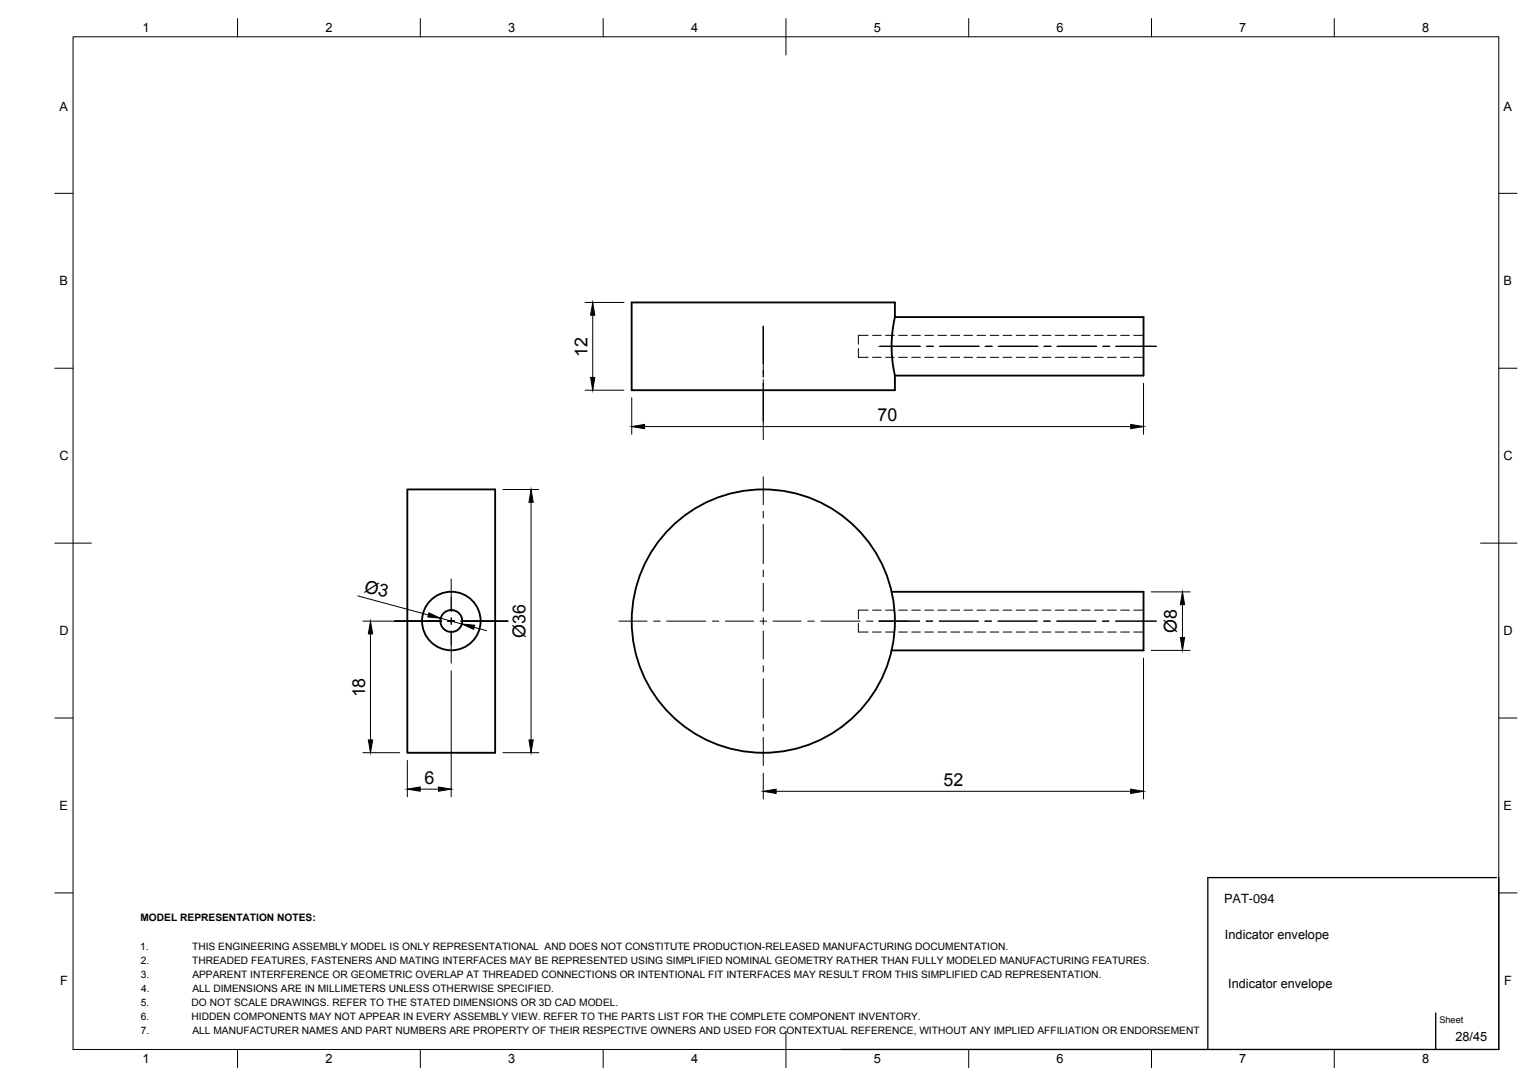
ISO-10303-21;
HEADER;
/* Generated by software containing ST-Developer
 * from STEP Tools, Inc. (www.steptools.com) 
 */

FILE_DESCRIPTION(
/* description */ ('Shaft runout checking stand'),
/* implementation_level */ '2;1');

FILE_NAME(
/* name */ 'Indicator envelope.step',
/* time_stamp */ '2026-11-02T21:12:33-08:00',
/* author */ (''),
/* organization */ (''),
/* preprocessor_version */ 'ST-DEVELOPER v20.2',
/* originating_system */ 'Autodesk Translation Framework v15.17.0.0',
/* authorisation */ '');

FILE_SCHEMA (('AUTOMOTIVE_DESIGN { 1 0 10303 214 3 1 1 }'));
ENDSEC;

DATA;
#10=MECHANICAL_DESIGN_GEOMETRIC_PRESENTATION_REPRESENTATION('',(#490),#11748);
#333=B_SPLINE_CURVE_WITH_KNOTS('',3,(#10807,#10808,#10809,#10810,#10811,
#10812,#10813,#10814,#10815,#10816,#10817,#10818,#10819,#10820,#10821,#10822,
#10823,#10824),.UNSPECIFIED.,.F.,.F.,(4,2,2,2,2,2,2,2,4),(0.,0.151225950236217,
0.302451900472435,0.453664817813398,0.604877735154361,0.756090652495325,
0.907303569836288,1.05852952007251,1.20975547030872),.UNSPECIFIED.);
#334=B_SPLINE_CURVE_WITH_KNOTS('',3,(#10825,#10826,#10827,#10828,#10829,
#10830,#10831,#10832,#10833,#10834,#10835,#10836,#10837,#10838,#10839,#10840,
#10841,#10842),.UNSPECIFIED.,.F.,.F.,(4,2,2,2,2,2,2,2,4),(1.20975547030872,
1.36098142054494,1.51220737078116,1.66342028812212,1.81463320546308,1.96584612280405,
2.11705904014501,2.26828499038123,2.41951094061745),.UNSPECIFIED.);
#404=SHAPE_REPRESENTATION_RELATIONSHIP('SRR','None',#11953,#447);
#447=ADVANCED_BREP_SHAPE_REPRESENTATION('',(#538),#11729);
#490=STYLED_ITEM('',(#12169),#538);
#538=MANIFOLD_SOLID_BREP('Body1',#6236);
#650=FACE_BOUND('',#1770,.T.);
#651=FACE_BOUND('',#1772,.T.);
#831=CIRCLE('',#7197,0.15);
#832=CIRCLE('',#7198,0.15);
#833=CIRCLE('',#7201,0.4);
#834=CIRCLE('',#7204,1.8);
#835=CIRCLE('',#7205,1.8);
#1008=CYLINDRICAL_SURFACE('',#7196,0.15);
#1009=CYLINDRICAL_SURFACE('',#7200,0.4);
#1010=CYLINDRICAL_SURFACE('',#7203,1.8);
#1310=FACE_OUTER_BOUND('',#1766,.T.);
#1311=FACE_OUTER_BOUND('',#1767,.T.);
#1312=FACE_OUTER_BOUND('',#1768,.T.);
#1313=FACE_OUTER_BOUND('',#1769,.T.);
#1314=FACE_OUTER_BOUND('',#1771,.T.);
#1315=FACE_OUTER_BOUND('',#1773,.T.);
#1316=FACE_OUTER_BOUND('',#1774,.T.);
#1766=EDGE_LOOP('',(#5264,#5265,#5266,#5267));
#1767=EDGE_LOOP('',(#5268));
#1768=EDGE_LOOP('',(#5269,#5270,#5271,#5272,#5273));
#1769=EDGE_LOOP('',(#5274));
#1770=EDGE_LOOP('',(#5275));
#1771=EDGE_LOOP('',(#5276,#5277,#5278,#5279));
#1772=EDGE_LOOP('',(#5280,#5281));
#1773=EDGE_LOOP('',(#5282));
#1774=EDGE_LOOP('',(#5283));
#2309=LINE('',#10801,#2776);
#2310=LINE('',#10844,#2777);
#2311=LINE('',#10851,#2778);
#2776=VECTOR('',#8844,0.15);
#2777=VECTOR('',#8851,0.4);
#2778=VECTOR('',#8860,1.8);
#3207=VERTEX_POINT('',#10798);
#3208=VERTEX_POINT('',#10800);
#3209=VERTEX_POINT('',#10805);
#3210=VERTEX_POINT('',#10806);
#3211=VERTEX_POINT('',#10843);
#3212=VERTEX_POINT('',#10848);
#3213=VERTEX_POINT('',#10850);
#3918=EDGE_CURVE('',#3207,#3207,#831,.T.);
#3919=EDGE_CURVE('',#3207,#3208,#2309,.T.);
#3920=EDGE_CURVE('',#3208,#3208,#832,.T.);
#3921=EDGE_CURVE('',#3209,#3210,#333,.T.);
#3922=EDGE_CURVE('',#3210,#3209,#334,.T.);
#3923=EDGE_CURVE('',#3210,#3211,#2310,.T.);
#3924=EDGE_CURVE('',#3211,#3211,#833,.T.);
#3925=EDGE_CURVE('',#3212,#3212,#834,.T.);
#3926=EDGE_CURVE('',#3212,#3213,#2311,.T.);
#3927=EDGE_CURVE('',#3213,#3213,#835,.T.);
#5264=ORIENTED_EDGE('',*,*,#3918,.F.);
#5265=ORIENTED_EDGE('',*,*,#3919,.T.);
#5266=ORIENTED_EDGE('',*,*,#3920,.T.);
#5267=ORIENTED_EDGE('',*,*,#3919,.F.);
#5268=ORIENTED_EDGE('',*,*,#3920,.F.);
#5269=ORIENTED_EDGE('',*,*,#3921,.F.);
#5270=ORIENTED_EDGE('',*,*,#3922,.F.);
#5271=ORIENTED_EDGE('',*,*,#3923,.T.);
#5272=ORIENTED_EDGE('',*,*,#3924,.T.);
#5273=ORIENTED_EDGE('',*,*,#3923,.F.);
#5274=ORIENTED_EDGE('',*,*,#3924,.F.);
#5275=ORIENTED_EDGE('',*,*,#3918,.T.);
#5276=ORIENTED_EDGE('',*,*,#3925,.F.);
#5277=ORIENTED_EDGE('',*,*,#3926,.T.);
#5278=ORIENTED_EDGE('',*,*,#3927,.T.);
#5279=ORIENTED_EDGE('',*,*,#3926,.F.);
#5280=ORIENTED_EDGE('',*,*,#3921,.T.);
#5281=ORIENTED_EDGE('',*,*,#3922,.T.);
#5282=ORIENTED_EDGE('',*,*,#3925,.T.);
#5283=ORIENTED_EDGE('',*,*,#3927,.F.);
#5794=PLANE('',#7199);
#5795=PLANE('',#7202);
#5796=PLANE('',#7206);
#5797=PLANE('',#7207);
#6110=ADVANCED_FACE('',(#1310),#1008,.F.);
#6111=ADVANCED_FACE('',(#1311),#5794,.F.);
#6112=ADVANCED_FACE('',(#1312),#1009,.T.);
#6113=ADVANCED_FACE('',(#1313,#650),#5795,.F.);
#6114=ADVANCED_FACE('',(#1314,#651),#1010,.T.);
#6115=ADVANCED_FACE('',(#1315),#5796,.T.);
#6116=ADVANCED_FACE('',(#1316),#5797,.F.);
#6236=CLOSED_SHELL('',(#6110,#6111,#6112,#6113,#6114,#6115,#6116));
#7195=AXIS2_PLACEMENT_3D('',#10796,#8838,#8839);
#7196=AXIS2_PLACEMENT_3D('',#10797,#8840,#8841);
#7197=AXIS2_PLACEMENT_3D('',#10799,#8842,#8843);
#7198=AXIS2_PLACEMENT_3D('',#10802,#8845,#8846);
#7199=AXIS2_PLACEMENT_3D('',#10803,#8847,#8848);
#7200=AXIS2_PLACEMENT_3D('',#10804,#8849,#8850);
#7201=AXIS2_PLACEMENT_3D('',#10845,#8852,#8853);
#7202=AXIS2_PLACEMENT_3D('',#10846,#8854,#8855);
#7203=AXIS2_PLACEMENT_3D('',#10847,#8856,#8857);
#7204=AXIS2_PLACEMENT_3D('',#10849,#8858,#8859);
#7205=AXIS2_PLACEMENT_3D('',#10852,#8861,#8862);
#7206=AXIS2_PLACEMENT_3D('',#10853,#8863,#8864);
#7207=AXIS2_PLACEMENT_3D('',#10854,#8865,#8866);
#8838=DIRECTION('axis',(0.,0.,1.));
#8839=DIRECTION('refdir',(1.,0.,0.));
#8840=DIRECTION('center_axis',(0.,0.,1.));
#8841=DIRECTION('ref_axis',(1.,0.,0.));
#8842=DIRECTION('center_axis',(0.,0.,1.));
#8843=DIRECTION('ref_axis',(1.,0.,0.));
#8844=DIRECTION('',(0.,0.,1.));
#8845=DIRECTION('center_axis',(0.,0.,1.));
#8846=DIRECTION('ref_axis',(1.,0.,0.));
#8847=DIRECTION('center_axis',(0.,0.,1.));
#8848=DIRECTION('ref_axis',(1.,0.,0.));
#8849=DIRECTION('center_axis',(0.,0.,1.));
#8850=DIRECTION('ref_axis',(1.,0.,0.));
#8851=DIRECTION('',(0.,0.,-1.));
#8852=DIRECTION('center_axis',(0.,0.,1.));
#8853=DIRECTION('ref_axis',(1.,0.,0.));
#8854=DIRECTION('center_axis',(0.,0.,1.));
#8855=DIRECTION('ref_axis',(1.,0.,0.));
#8856=DIRECTION('center_axis',(0.,1.,0.));
#8857=DIRECTION('ref_axis',(1.,0.,0.));
#8858=DIRECTION('center_axis',(0.,1.,0.));
#8859=DIRECTION('ref_axis',(1.,0.,0.));
#8860=DIRECTION('',(0.,-1.,0.));
#8861=DIRECTION('center_axis',(0.,1.,0.));
#8862=DIRECTION('ref_axis',(1.,0.,0.));
#8863=DIRECTION('center_axis',(0.,1.,0.));
#8864=DIRECTION('ref_axis',(1.,0.,0.));
#8865=DIRECTION('center_axis',(0.,1.,0.));
#8866=DIRECTION('ref_axis',(1.,0.,0.));
#10796=CARTESIAN_POINT('',(0.,0.,0.));
#10797=CARTESIAN_POINT('Origin',(0.,0.,9.9));
#10798=CARTESIAN_POINT('',(-0.15,-1.83697019872103E-17,10.));
#10799=CARTESIAN_POINT('Origin',(0.,0.,10.));
#10800=CARTESIAN_POINT('',(-0.15,-1.83697019872103E-17,13.9));
#10801=CARTESIAN_POINT('',(-0.15,-1.83697019872103E-17,9.9));
#10802=CARTESIAN_POINT('Origin',(0.,0.,13.9));
#10803=CARTESIAN_POINT('Origin',(0.,0.,13.9));
#10804=CARTESIAN_POINT('Origin',(0.,0.,10.));
#10805=CARTESIAN_POINT('',(0.4,-4.16333634234434E-17,13.4450071225216));
#10806=CARTESIAN_POINT('',(-0.4,-4.89858719658941E-17,13.4450071225216));
#10807=CARTESIAN_POINT('Ctrl Pts',(0.4,-4.16333634234434E-17,13.4450071225216));
#10808=CARTESIAN_POINT('Ctrl Pts',(0.4,0.0504086500787391,13.4450071225216));
#10809=CARTESIAN_POINT('Ctrl Pts',(0.389891257329757,0.10405747970835,13.4426096554494));
#10810=CARTESIAN_POINT('Ctrl Pts',(0.349018656101199,0.202556511873035,
13.4340379438059));
#10811=CARTESIAN_POINT('Ctrl Pts',(0.318263533348268,0.24742189160097,13.4279969749484));
#10812=CARTESIAN_POINT('Ctrl Pts',(0.247424944224197,0.318260480725041,
13.4167257438327));
#10813=CARTESIAN_POINT('Ctrl Pts',(0.202558278587653,0.349017990321186,
13.4107505468858));
#10814=CARTESIAN_POINT('Ctrl Pts',(0.104054739507664,0.389892327061432,
13.4023303772031));
#10815=CARTESIAN_POINT('Ctrl Pts',(0.0504043057803212,0.4,13.4));
#10816=CARTESIAN_POINT('Ctrl Pts',(-0.0504043057803211,0.4,13.4));
#10817=CARTESIAN_POINT('Ctrl Pts',(-0.104054739507664,0.389892327061432,
13.4023303772031));
#10818=CARTESIAN_POINT('Ctrl Pts',(-0.202558278587653,0.349017990321186,
13.4107505468858));
#10819=CARTESIAN_POINT('Ctrl Pts',(-0.247424944224197,0.318260480725041,
13.4167257438327));
#10820=CARTESIAN_POINT('Ctrl Pts',(-0.318263533348268,0.24742189160097,
13.4279969749484));
#10821=CARTESIAN_POINT('Ctrl Pts',(-0.349018656101199,0.202556511873035,
13.4340379438059));
#10822=CARTESIAN_POINT('Ctrl Pts',(-0.389891257329757,0.10405747970835,
13.4426096554494));
#10823=CARTESIAN_POINT('Ctrl Pts',(-0.4,0.0504086500787392,13.4450071225216));
#10824=CARTESIAN_POINT('Ctrl Pts',(-0.4,1.38777878078145E-17,13.4450071225216));
#10825=CARTESIAN_POINT('Ctrl Pts',(-0.4,5.55111512312578E-17,13.4450071225216));
#10826=CARTESIAN_POINT('Ctrl Pts',(-0.4,-0.0504086500787391,13.4450071225216));
#10827=CARTESIAN_POINT('Ctrl Pts',(-0.389891257329757,-0.10405747970835,
13.4426096554494));
#10828=CARTESIAN_POINT('Ctrl Pts',(-0.349018656101199,-0.202556511873035,
13.4340379438059));
#10829=CARTESIAN_POINT('Ctrl Pts',(-0.318263533348268,-0.24742189160097,
13.4279969749484));
#10830=CARTESIAN_POINT('Ctrl Pts',(-0.247424944224197,-0.318260480725041,
13.4167257438327));
#10831=CARTESIAN_POINT('Ctrl Pts',(-0.202558278587653,-0.349017990321186,
13.4107505468858));
#10832=CARTESIAN_POINT('Ctrl Pts',(-0.104054739507664,-0.389892327061432,
13.4023303772031));
#10833=CARTESIAN_POINT('Ctrl Pts',(-0.0504043057803212,-0.4,13.4));
#10834=CARTESIAN_POINT('Ctrl Pts',(0.050404305780321,-0.4,13.4));
#10835=CARTESIAN_POINT('Ctrl Pts',(0.104054739507664,-0.389892327061432,
13.4023303772031));
#10836=CARTESIAN_POINT('Ctrl Pts',(0.202558278587653,-0.349017990321186,
13.4107505468858));
#10837=CARTESIAN_POINT('Ctrl Pts',(0.247424944224197,-0.318260480725041,
13.4167257438327));
#10838=CARTESIAN_POINT('Ctrl Pts',(0.318263533348268,-0.24742189160097,
13.4279969749484));
#10839=CARTESIAN_POINT('Ctrl Pts',(0.349018656101199,-0.202556511873035,
13.4340379438059));
#10840=CARTESIAN_POINT('Ctrl Pts',(0.389891257329757,-0.10405747970835,
13.4426096554494));
#10841=CARTESIAN_POINT('Ctrl Pts',(0.4,-0.0504086500787392,13.4450071225216));
#10842=CARTESIAN_POINT('Ctrl Pts',(0.4,-1.38777878078145E-17,13.4450071225216));
#10843=CARTESIAN_POINT('',(-0.4,-4.89858719658941E-17,10.));
#10844=CARTESIAN_POINT('',(-0.4,-4.89858719658941E-17,10.));
#10845=CARTESIAN_POINT('Origin',(0.,0.,10.));
#10846=CARTESIAN_POINT('Origin',(0.,0.,10.));
#10847=CARTESIAN_POINT('Origin',(0.,-0.6,15.2));
#10848=CARTESIAN_POINT('',(-1.8,0.6,15.2));
#10849=CARTESIAN_POINT('Origin',(0.,0.6,15.2));
#10850=CARTESIAN_POINT('',(-1.8,-0.6,15.2));
#10851=CARTESIAN_POINT('',(-1.8,-0.6,15.2));
#10852=CARTESIAN_POINT('Origin',(0.,-0.6,15.2));
#10853=CARTESIAN_POINT('Origin',(0.,0.6,15.2));
#10854=CARTESIAN_POINT('Origin',(0.,-0.6,15.2));
#11680=UNCERTAINTY_MEASURE_WITH_UNIT(LENGTH_MEASURE(0.001),#11749,
'DISTANCE_ACCURACY_VALUE',
'Maximum model space distance between geometric entities at asserted c
onnectivities');
#11699=UNCERTAINTY_MEASURE_WITH_UNIT(LENGTH_MEASURE(0.001),#11749,
'DISTANCE_ACCURACY_VALUE',
'Maximum model space distance between geometric entities at asserted c
onnectivities');
#11729=(
GEOMETRIC_REPRESENTATION_CONTEXT(3)
GLOBAL_UNCERTAINTY_ASSIGNED_CONTEXT((#11680))
GLOBAL_UNIT_ASSIGNED_CONTEXT((#11749,#11751,#11752))
REPRESENTATION_CONTEXT('','3D')
);
#11748=(
GEOMETRIC_REPRESENTATION_CONTEXT(3)
GLOBAL_UNCERTAINTY_ASSIGNED_CONTEXT((#11699))
GLOBAL_UNIT_ASSIGNED_CONTEXT((#11749,#11751,#11752))
REPRESENTATION_CONTEXT('','3D')
);
#11749=(
LENGTH_UNIT()
NAMED_UNIT(*)
SI_UNIT(.CENTI.,.METRE.)
);
#11751=(
NAMED_UNIT(*)
PLANE_ANGLE_UNIT()
SI_UNIT($,.RADIAN.)
);
#11752=(
NAMED_UNIT(*)
SI_UNIT($,.STERADIAN.)
SOLID_ANGLE_UNIT()
);
#11782=SHAPE_DEFINITION_REPRESENTATION(#11830,#11953);
#11830=PRODUCT_DEFINITION_SHAPE('',$,#12002);
#11953=SHAPE_REPRESENTATION('',(#7195),#11729);
#11972=PRODUCT_DEFINITION_CONTEXT('part definition',#12118,'design');
#12002=PRODUCT_DEFINITION('Indicator envelope','Indicator envelope',#12050,
#11972);
#12050=PRODUCT_DEFINITION_FORMATION('',$,#12149);
#12118=APPLICATION_CONTEXT(
'Core Data for Automotive Mechanical Design Process');
#12119=PRODUCT_CONTEXT('part definition',#12118,'mechanical');
#12149=PRODUCT('Indicator envelope','Indicator envelope',
'Indicator envelope',(#12119));
#12169=PRESENTATION_STYLE_ASSIGNMENT((#12174));
#12174=SURFACE_STYLE_USAGE(.BOTH.,#12179);
#12179=SURFACE_SIDE_STYLE('',(#12184));
#12184=SURFACE_STYLE_FILL_AREA(#12189);
#12189=FILL_AREA_STYLE('CAD Library Painted - Engineering blue',(#12194));
#12194=FILL_AREA_STYLE_COLOUR('CAD Library Painted - Engineering blue',
#12199);
#12199=COLOUR_RGB('CAD Library Painted - Engineering blue',0.12156862745098,
0.356862745098039,0.6);
ENDSEC;
END-ISO-10303-21;
